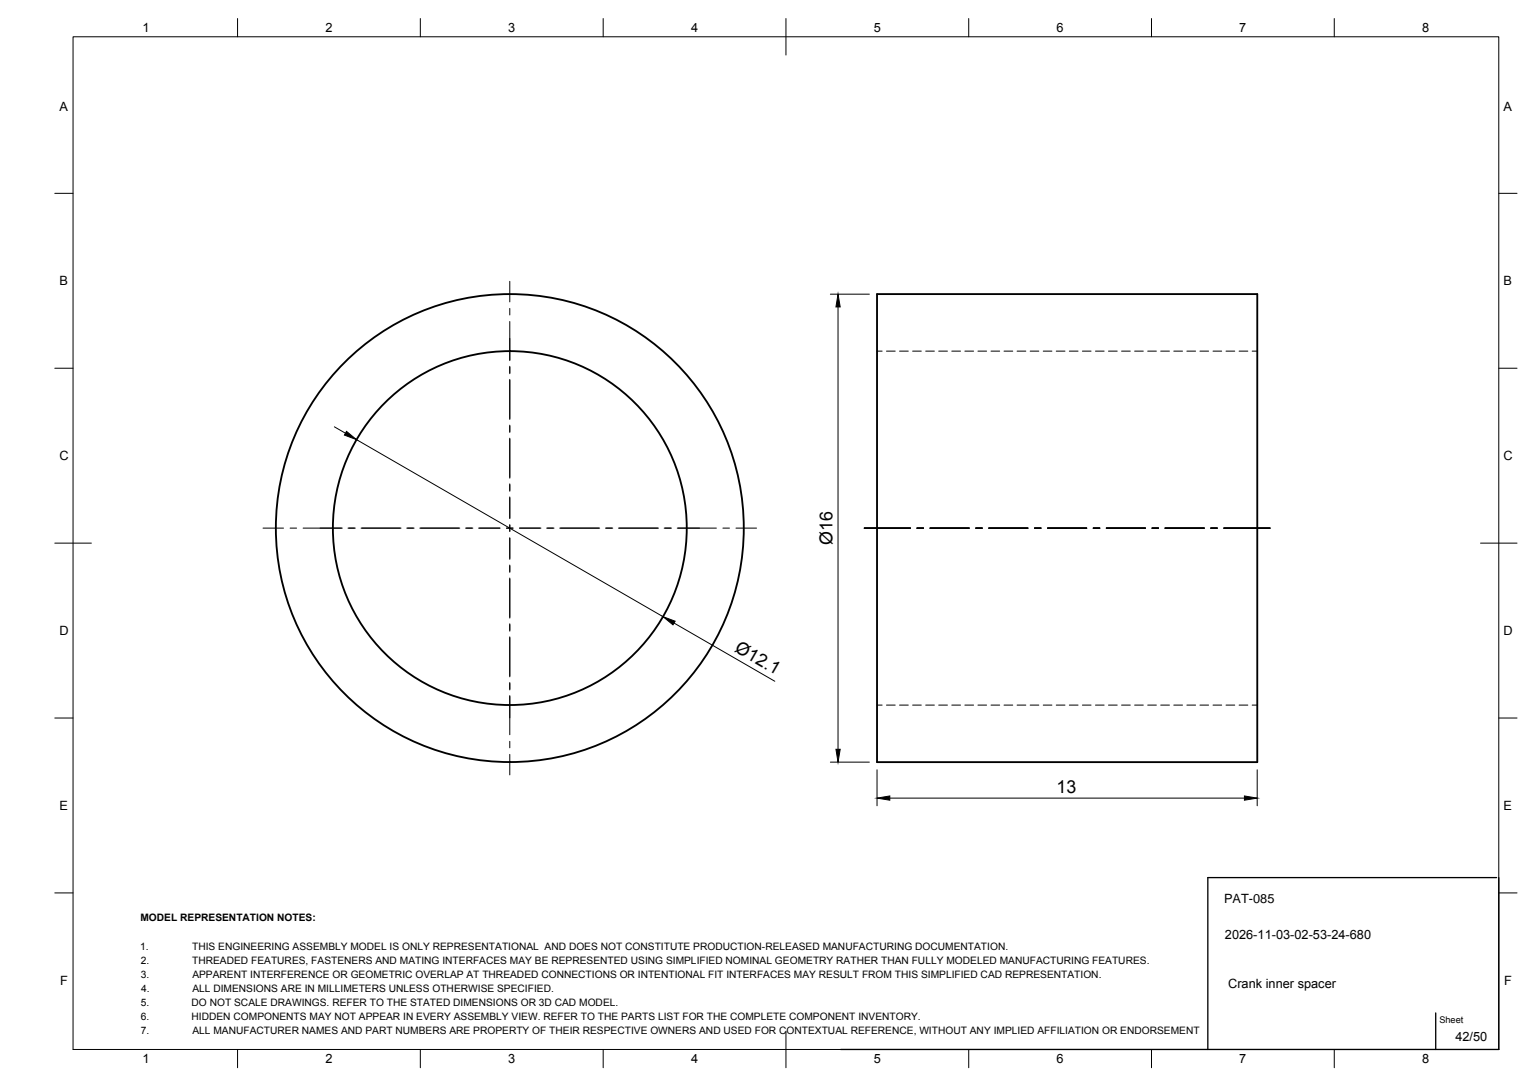
ISO-10303-21;
HEADER;
/* Generated by software containing ST-Developer
 * from STEP Tools, Inc. (www.steptools.com) 
 */

FILE_DESCRIPTION(
/* description */ ('Rack and pinion manual slide'),
/* implementation_level */ '2;1');

FILE_NAME(
/* name */ 'Crank inner spacer.step',
/* time_stamp */ '2026-10-28T03:22:49-07:00',
/* author */ (''),
/* organization */ (''),
/* preprocessor_version */ 'ST-DEVELOPER v20.2',
/* originating_system */ 'Autodesk Translation Framework v15.17.0.0',
/* authorisation */ '');

FILE_SCHEMA (('AUTOMOTIVE_DESIGN { 1 0 10303 214 3 1 1 }'));
ENDSEC;

DATA;
#10=MECHANICAL_DESIGN_GEOMETRIC_PRESENTATION_REPRESENTATION('',(#773),#34851);
#674=SHAPE_REPRESENTATION_RELATIONSHIP('SRR','None',#35113,#720);
#720=ADVANCED_BREP_SHAPE_REPRESENTATION('',(#823),#34838);
#773=STYLED_ITEM('',(#35404),#823);
#823=MANIFOLD_SOLID_BREP('Body1',#13796);
#1020=FACE_BOUND('',#3030,.T.);
#1021=FACE_BOUND('',#3032,.T.);
#1454=PLANE('',#15260);
#1455=PLANE('',#15261);
#2101=FACE_OUTER_BOUND('',#3027,.T.);
#2102=FACE_OUTER_BOUND('',#3028,.T.);
#2103=FACE_OUTER_BOUND('',#3029,.T.);
#2104=FACE_OUTER_BOUND('',#3031,.T.);
#3027=EDGE_LOOP('',(#12014,#12015,#12016,#12017));
#3028=EDGE_LOOP('',(#12018,#12019,#12020,#12021));
#3029=EDGE_LOOP('',(#12022));
#3030=EDGE_LOOP('',(#12023));
#3031=EDGE_LOOP('',(#12024));
#3032=EDGE_LOOP('',(#12025));
#4278=LINE('',#22691,#5569);
#4279=LINE('',#22697,#5570);
#5569=VECTOR('',#18532,0.605);
#5570=VECTOR('',#18539,0.800000000000001);
#6126=CIRCLE('',#15255,0.605);
#6127=CIRCLE('',#15256,0.605);
#6128=CIRCLE('',#15258,0.800000000000001);
#6129=CIRCLE('',#15259,0.800000000000001);
#7155=VERTEX_POINT('',#22688);
#7156=VERTEX_POINT('',#22690);
#7157=VERTEX_POINT('',#22694);
#7158=VERTEX_POINT('',#22696);
#8819=EDGE_CURVE('',#7155,#7155,#6126,.T.);
#8820=EDGE_CURVE('',#7155,#7156,#4278,.T.);
#8821=EDGE_CURVE('',#7156,#7156,#6127,.T.);
#8822=EDGE_CURVE('',#7157,#7157,#6128,.T.);
#8823=EDGE_CURVE('',#7157,#7158,#4279,.T.);
#8824=EDGE_CURVE('',#7158,#7158,#6129,.T.);
#12014=ORIENTED_EDGE('',*,*,#8819,.F.);
#12015=ORIENTED_EDGE('',*,*,#8820,.T.);
#12016=ORIENTED_EDGE('',*,*,#8821,.T.);
#12017=ORIENTED_EDGE('',*,*,#8820,.F.);
#12018=ORIENTED_EDGE('',*,*,#8822,.F.);
#12019=ORIENTED_EDGE('',*,*,#8823,.T.);
#12020=ORIENTED_EDGE('',*,*,#8824,.T.);
#12021=ORIENTED_EDGE('',*,*,#8823,.F.);
#12022=ORIENTED_EDGE('',*,*,#8822,.T.);
#12023=ORIENTED_EDGE('',*,*,#8819,.T.);
#12024=ORIENTED_EDGE('',*,*,#8824,.F.);
#12025=ORIENTED_EDGE('',*,*,#8821,.F.);
#12969=CYLINDRICAL_SURFACE('',#15254,0.605);
#12970=CYLINDRICAL_SURFACE('',#15257,0.800000000000001);
#13579=ADVANCED_FACE('',(#2101),#12969,.F.);
#13580=ADVANCED_FACE('',(#2102),#12970,.T.);
#13581=ADVANCED_FACE('',(#2103,#1020),#1454,.T.);
#13582=ADVANCED_FACE('',(#2104,#1021),#1455,.F.);
#13796=CLOSED_SHELL('',(#13579,#13580,#13581,#13582));
#15253=AXIS2_PLACEMENT_3D('',#22686,#18526,#18527);
#15254=AXIS2_PLACEMENT_3D('',#22687,#18528,#18529);
#15255=AXIS2_PLACEMENT_3D('',#22689,#18530,#18531);
#15256=AXIS2_PLACEMENT_3D('',#22692,#18533,#18534);
#15257=AXIS2_PLACEMENT_3D('',#22693,#18535,#18536);
#15258=AXIS2_PLACEMENT_3D('',#22695,#18537,#18538);
#15259=AXIS2_PLACEMENT_3D('',#22698,#18540,#18541);
#15260=AXIS2_PLACEMENT_3D('',#22699,#18542,#18543);
#15261=AXIS2_PLACEMENT_3D('',#22700,#18544,#18545);
#18526=DIRECTION('axis',(0.,0.,1.));
#18527=DIRECTION('refdir',(1.,0.,0.));
#18528=DIRECTION('center_axis',(0.,1.,0.));
#18529=DIRECTION('ref_axis',(1.,0.,0.));
#18530=DIRECTION('center_axis',(0.,-1.,0.));
#18531=DIRECTION('ref_axis',(1.,0.,0.));
#18532=DIRECTION('',(0.,-1.,0.));
#18533=DIRECTION('center_axis',(0.,-1.,0.));
#18534=DIRECTION('ref_axis',(1.,0.,0.));
#18535=DIRECTION('center_axis',(0.,1.,0.));
#18536=DIRECTION('ref_axis',(1.,0.,0.));
#18537=DIRECTION('center_axis',(0.,1.,0.));
#18538=DIRECTION('ref_axis',(1.,0.,0.));
#18539=DIRECTION('',(0.,-1.,0.));
#18540=DIRECTION('center_axis',(0.,1.,0.));
#18541=DIRECTION('ref_axis',(1.,0.,0.));
#18542=DIRECTION('center_axis',(0.,1.,0.));
#18543=DIRECTION('ref_axis',(1.,0.,0.));
#18544=DIRECTION('center_axis',(0.,1.,0.));
#18545=DIRECTION('ref_axis',(1.,0.,0.));
#22686=CARTESIAN_POINT('',(0.,0.,0.));
#22687=CARTESIAN_POINT('Origin',(11.,4.7,10.25));
#22688=CARTESIAN_POINT('',(10.395,6.,10.25));
#22689=CARTESIAN_POINT('Origin',(11.,6.,10.25));
#22690=CARTESIAN_POINT('',(10.395,4.7,10.25));
#22691=CARTESIAN_POINT('',(10.395,4.7,10.25));
#22692=CARTESIAN_POINT('Origin',(11.,4.7,10.25));
#22693=CARTESIAN_POINT('Origin',(11.,4.7,10.25));
#22694=CARTESIAN_POINT('',(10.2,6.,10.25));
#22695=CARTESIAN_POINT('Origin',(11.,6.,10.25));
#22696=CARTESIAN_POINT('',(10.2,4.7,10.25));
#22697=CARTESIAN_POINT('',(10.2,4.7,10.25));
#22698=CARTESIAN_POINT('Origin',(11.,4.7,10.25));
#22699=CARTESIAN_POINT('Origin',(11.,6.,10.25));
#22700=CARTESIAN_POINT('Origin',(11.,4.7,10.25));
#34784=UNCERTAINTY_MEASURE_WITH_UNIT(LENGTH_MEASURE(0.001),#34852,
'DISTANCE_ACCURACY_VALUE',
'Maximum model space distance between geometric entities at asserted c
onnectivities');
#34797=UNCERTAINTY_MEASURE_WITH_UNIT(LENGTH_MEASURE(0.001),#34852,
'DISTANCE_ACCURACY_VALUE',
'Maximum model space distance between geometric entities at asserted c
onnectivities');
#34838=(
GEOMETRIC_REPRESENTATION_CONTEXT(3)
GLOBAL_UNCERTAINTY_ASSIGNED_CONTEXT((#34784))
GLOBAL_UNIT_ASSIGNED_CONTEXT((#34852,#34854,#34855))
REPRESENTATION_CONTEXT('','3D')
);
#34851=(
GEOMETRIC_REPRESENTATION_CONTEXT(3)
GLOBAL_UNCERTAINTY_ASSIGNED_CONTEXT((#34797))
GLOBAL_UNIT_ASSIGNED_CONTEXT((#34852,#34854,#34855))
REPRESENTATION_CONTEXT('','3D')
);
#34852=(
LENGTH_UNIT()
NAMED_UNIT(*)
SI_UNIT(.CENTI.,.METRE.)
);
#34854=(
NAMED_UNIT(*)
PLANE_ANGLE_UNIT()
SI_UNIT($,.RADIAN.)
);
#34855=(
NAMED_UNIT(*)
SI_UNIT($,.STERADIAN.)
SOLID_ANGLE_UNIT()
);
#34896=SHAPE_DEFINITION_REPRESENTATION(#34957,#35113);
#34957=PRODUCT_DEFINITION_SHAPE('',$,#35167);
#35113=SHAPE_REPRESENTATION('',(#15253),#34838);
#35126=PRODUCT_DEFINITION_CONTEXT('part definition',#35287,'design');
#35167=PRODUCT_DEFINITION('Crank inner spacer','Crank inner spacer',#35220,
#35126);
#35220=PRODUCT_DEFINITION_FORMATION('',$,#35329);
#35287=APPLICATION_CONTEXT(
'Core Data for Automotive Mechanical Design Process');
#35288=PRODUCT_CONTEXT('part definition',#35287,'mechanical');
#35329=PRODUCT('Crank inner spacer','Crank inner spacer',
'Crank inner spacer',(#35288));
#35398=COLOUR_RGB('Sky Blue',0.24,0.69,0.87);
#35399=FILL_AREA_STYLE_COLOUR('',#35398);
#35400=FILL_AREA_STYLE('',(#35399));
#35401=SURFACE_STYLE_FILL_AREA(#35400);
#35402=SURFACE_SIDE_STYLE('',(#35401));
#35403=SURFACE_STYLE_USAGE(.BOTH.,#35402);
#35404=PRESENTATION_STYLE_ASSIGNMENT((#35403));
ENDSEC;
END-ISO-10303-21;
